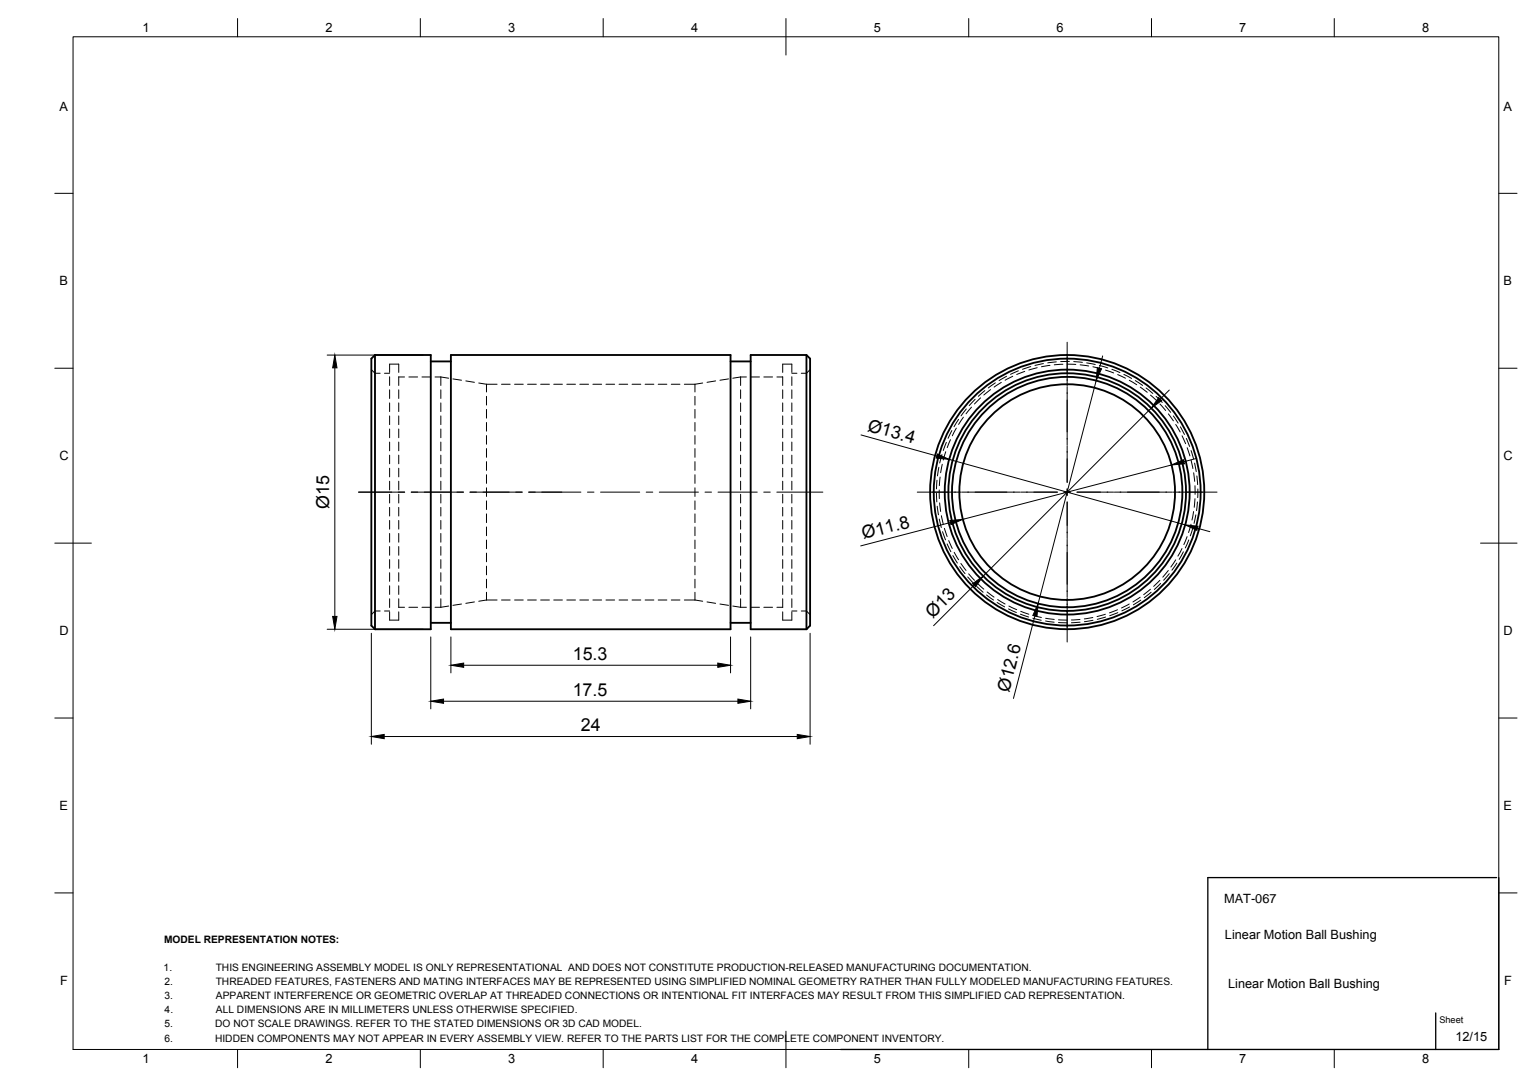
ISO-10303-21;
HEADER;
/* Generated by software containing ST-Developer
 * from STEP Tools, Inc. (www.steptools.com) 
 */

FILE_DESCRIPTION(
/* description */ ('CAx-IF Rec.Pracs.---Representation and Presentation of Product Manufa
cturing Information (PMI)---4.0---2014-10-13'),
/* implementation_level */ '2;1');

FILE_NAME(
/* name */ 'Linear Motion Ball Bushing.step',
/* time_stamp */ '2026-10-24T16:02:03-07:00',
/* author */ (''),
/* organization */ (''),
/* preprocessor_version */ 'ST-DEVELOPER v20.2',
/* originating_system */ 'Autodesk Translation Framework v15.17.0.0',
/* authorisation */ '');

FILE_SCHEMA (('AP242_MANAGED_MODEL_BASED_3D_ENGINEERING_MIM_LF { 1 0 10303 442 2 1 4 }'));
ENDSEC;

DATA;
#10=MECHANICAL_DESIGN_GEOMETRIC_PRESENTATION_REPRESENTATION('',(#356),#6348);
#315=CONICAL_SURFACE('',#3805,0.0066,0.785398163397459);
#316=CONICAL_SURFACE('',#3813,0.0074,0.785398163397448);
#317=CONICAL_SURFACE('',#3818,0.0066,0.785398163397459);
#318=CONICAL_SURFACE('',#3826,0.0074,0.785398163397448);
#319=CONICAL_SURFACE('',#3839,0.0061,0.158655262186402);
#320=CONICAL_SURFACE('',#3843,0.0061,0.158655262186402);
#334=SHAPE_REPRESENTATION_RELATIONSHIP('SRR','None',#6496,#345);
#345=ADVANCED_BREP_SHAPE_REPRESENTATION('',(#367),#6344);
#356=STYLED_ITEM('',(#6603),#367);
#367=MANIFOLD_SOLID_BREP('Body1',#3395);
#446=CYLINDRICAL_SURFACE('',#3811,0.0065);
#447=CYLINDRICAL_SURFACE('',#3816,0.0075);
#448=CYLINDRICAL_SURFACE('',#3824,0.0065);
#449=CYLINDRICAL_SURFACE('',#3829,0.0075);
#450=CYLINDRICAL_SURFACE('',#3833,0.00700000010430813);
#451=CYLINDRICAL_SURFACE('',#3837,0.0063);
#452=CYLINDRICAL_SURFACE('',#3841,0.0059);
#453=CYLINDRICAL_SURFACE('',#3845,0.0063);
#454=CYLINDRICAL_SURFACE('',#3849,0.00700000010430813);
#455=CYLINDRICAL_SURFACE('',#3854,0.00715);
#456=CYLINDRICAL_SURFACE('',#3858,0.0075);
#457=CYLINDRICAL_SURFACE('',#3862,0.00715);
#488=FACE_BOUND('',#1016,.T.);
#489=FACE_BOUND('',#1022,.T.);
#490=FACE_BOUND('',#1027,.T.);
#491=FACE_BOUND('',#1030,.T.);
#492=FACE_BOUND('',#1037,.T.);
#493=FACE_BOUND('',#1040,.T.);
#494=FACE_BOUND('',#1042,.T.);
#495=FACE_BOUND('',#1045,.T.);
#496=FACE_BOUND('',#1048,.T.);
#497=FACE_BOUND('',#1051,.T.);
#644=CIRCLE('',#3806,0.00650000000001);
#645=CIRCLE('',#3807,0.00670000000001);
#646=CIRCLE('',#3808,0.00650000000001);
#647=CIRCLE('',#3810,0.00730000000001);
#648=CIRCLE('',#3812,0.00650000000001);
#649=CIRCLE('',#3814,0.00750000000001);
#650=CIRCLE('',#3815,0.00750000000001);
#651=CIRCLE('',#3817,0.00750000000001);
#652=CIRCLE('',#3819,0.00650000000001);
#653=CIRCLE('',#3820,0.00670000000001);
#654=CIRCLE('',#3821,0.00650000000001);
#655=CIRCLE('',#3823,0.00730000000001);
#656=CIRCLE('',#3825,0.00650000000001);
#657=CIRCLE('',#3827,0.00750000000001);
#658=CIRCLE('',#3828,0.00750000000001);
#659=CIRCLE('',#3830,0.00750000000001);
#660=CIRCLE('',#3832,0.00700000010431813);
#661=CIRCLE('',#3834,0.00700000010431813);
#662=CIRCLE('',#3836,0.00630000000001);
#663=CIRCLE('',#3838,0.00630000000001);
#664=CIRCLE('',#3840,0.00590000000001);
#665=CIRCLE('',#3842,0.00590000000001);
#666=CIRCLE('',#3844,0.00630000000001);
#667=CIRCLE('',#3846,0.00630000000001);
#668=CIRCLE('',#3848,0.00700000010431813);
#669=CIRCLE('',#3850,0.00700000010431813);
#670=CIRCLE('',#3853,0.00715000000001);
#671=CIRCLE('',#3855,0.00715000000001);
#672=CIRCLE('',#3857,0.00750000000001);
#673=CIRCLE('',#3859,0.00750000000001);
#674=CIRCLE('',#3861,0.00715000000001);
#675=CIRCLE('',#3863,0.00715000000001);
#819=FACE_OUTER_BOUND('',#1014,.T.);
#820=FACE_OUTER_BOUND('',#1015,.T.);
#821=FACE_OUTER_BOUND('',#1017,.T.);
#822=FACE_OUTER_BOUND('',#1018,.T.);
#823=FACE_OUTER_BOUND('',#1019,.T.);
#824=FACE_OUTER_BOUND('',#1020,.T.);
#825=FACE_OUTER_BOUND('',#1021,.T.);
#826=FACE_OUTER_BOUND('',#1023,.T.);
#827=FACE_OUTER_BOUND('',#1024,.T.);
#828=FACE_OUTER_BOUND('',#1025,.T.);
#829=FACE_OUTER_BOUND('',#1026,.T.);
#830=FACE_OUTER_BOUND('',#1028,.T.);
#831=FACE_OUTER_BOUND('',#1029,.T.);
#832=FACE_OUTER_BOUND('',#1031,.T.);
#833=FACE_OUTER_BOUND('',#1032,.T.);
#834=FACE_OUTER_BOUND('',#1033,.T.);
#835=FACE_OUTER_BOUND('',#1034,.T.);
#836=FACE_OUTER_BOUND('',#1035,.T.);
#837=FACE_OUTER_BOUND('',#1036,.T.);
#838=FACE_OUTER_BOUND('',#1038,.T.);
#839=FACE_OUTER_BOUND('',#1039,.T.);
#840=FACE_OUTER_BOUND('',#1041,.T.);
#841=FACE_OUTER_BOUND('',#1043,.T.);
#842=FACE_OUTER_BOUND('',#1044,.T.);
#843=FACE_OUTER_BOUND('',#1046,.T.);
#844=FACE_OUTER_BOUND('',#1047,.T.);
#845=FACE_OUTER_BOUND('',#1049,.T.);
#846=FACE_OUTER_BOUND('',#1050,.T.);
#1014=EDGE_LOOP('',(#2981,#2982,#2983,#2984,#2985));
#1015=EDGE_LOOP('',(#2986));
#1016=EDGE_LOOP('',(#2987));
#1017=EDGE_LOOP('',(#2988,#2989,#2990,#2991,#2992));
#1018=EDGE_LOOP('',(#2993,#2994,#2995,#2996,#2997));
#1019=EDGE_LOOP('',(#2998,#2999,#3000,#3001,#3002));
#1020=EDGE_LOOP('',(#3003,#3004,#3005,#3006,#3007));
#1021=EDGE_LOOP('',(#3008));
#1022=EDGE_LOOP('',(#3009));
#1023=EDGE_LOOP('',(#3010,#3011,#3012,#3013,#3014));
#1024=EDGE_LOOP('',(#3015,#3016,#3017,#3018,#3019));
#1025=EDGE_LOOP('',(#3020,#3021,#3022,#3023,#3024));
#1026=EDGE_LOOP('',(#3025));
#1027=EDGE_LOOP('',(#3026));
#1028=EDGE_LOOP('',(#3027,#3028,#3029,#3030));
#1029=EDGE_LOOP('',(#3031));
#1030=EDGE_LOOP('',(#3032));
#1031=EDGE_LOOP('',(#3033,#3034,#3035,#3036));
#1032=EDGE_LOOP('',(#3037,#3038,#3039,#3040));
#1033=EDGE_LOOP('',(#3041,#3042,#3043,#3044));
#1034=EDGE_LOOP('',(#3045,#3046,#3047,#3048));
#1035=EDGE_LOOP('',(#3049,#3050,#3051,#3052));
#1036=EDGE_LOOP('',(#3053));
#1037=EDGE_LOOP('',(#3054));
#1038=EDGE_LOOP('',(#3055,#3056,#3057,#3058));
#1039=EDGE_LOOP('',(#3059));
#1040=EDGE_LOOP('',(#3060));
#1041=EDGE_LOOP('',(#3061));
#1042=EDGE_LOOP('',(#3062));
#1043=EDGE_LOOP('',(#3063,#3064,#3065,#3066));
#1044=EDGE_LOOP('',(#3067));
#1045=EDGE_LOOP('',(#3068));
#1046=EDGE_LOOP('',(#3069,#3070,#3071,#3072));
#1047=EDGE_LOOP('',(#3073));
#1048=EDGE_LOOP('',(#3074));
#1049=EDGE_LOOP('',(#3075,#3076,#3077,#3078));
#1050=EDGE_LOOP('',(#3079));
#1051=EDGE_LOOP('',(#3080));
#1283=LINE('',#6051,#1516);
#1284=LINE('',#6059,#1517);
#1285=LINE('',#6065,#1518);
#1286=LINE('',#6070,#1519);
#1287=LINE('',#6076,#1520);
#1288=LINE('',#6085,#1521);
#1289=LINE('',#6090,#1522);
#1290=LINE('',#6094,#1523);
#1291=LINE('',#6102,#1524);
#1292=LINE('',#6109,#1525);
#1293=LINE('',#6113,#1526);
#1294=LINE('',#6117,#1527);
#1295=LINE('',#6120,#1528);
#1296=LINE('',#6125,#1529);
#1297=LINE('',#6132,#1530);
#1298=LINE('',#6140,#1531);
#1299=LINE('',#6147,#1532);
#1300=LINE('',#6154,#1533);
#1516=VECTOR('',#4757,0.0066);
#1517=VECTOR('',#4768,0.0065);
#1518=VECTOR('',#4775,0.0074);
#1519=VECTOR('',#4782,0.0075);
#1520=VECTOR('',#4787,0.0066);
#1521=VECTOR('',#4800,0.0065);
#1522=VECTOR('',#4805,0.0074);
#1523=VECTOR('',#4810,0.0075);
#1524=VECTOR('',#4821,0.00700000010430813);
#1525=VECTOR('',#4830,0.0063);
#1526=VECTOR('',#4835,0.0061);
#1527=VECTOR('',#4840,0.0059);
#1528=VECTOR('',#4843,0.0061);
#1529=VECTOR('',#4850,0.0063);
#1530=VECTOR('',#4859,0.00700000010430813);
#1531=VECTOR('',#4870,0.00715);
#1532=VECTOR('',#4879,0.0075);
#1533=VECTOR('',#4888,0.00715);
#1782=VERTEX_POINT('',#6047);
#1783=VERTEX_POINT('',#6048);
#1784=VERTEX_POINT('',#6050);
#1785=VERTEX_POINT('',#6055);
#1786=VERTEX_POINT('',#6058);
#1787=VERTEX_POINT('',#6062);
#1788=VERTEX_POINT('',#6063);
#1789=VERTEX_POINT('',#6068);
#1790=VERTEX_POINT('',#6072);
#1791=VERTEX_POINT('',#6073);
#1792=VERTEX_POINT('',#6075);
#1793=VERTEX_POINT('',#6080);
#1794=VERTEX_POINT('',#6083);
#1795=VERTEX_POINT('',#6087);
#1796=VERTEX_POINT('',#6088);
#1797=VERTEX_POINT('',#6093);
#1798=VERTEX_POINT('',#6097);
#1799=VERTEX_POINT('',#6100);
#1800=VERTEX_POINT('',#6104);
#1801=VERTEX_POINT('',#6107);
#1802=VERTEX_POINT('',#6111);
#1803=VERTEX_POINT('',#6115);
#1804=VERTEX_POINT('',#6119);
#1805=VERTEX_POINT('',#6123);
#1806=VERTEX_POINT('',#6127);
#1807=VERTEX_POINT('',#6130);
#1808=VERTEX_POINT('',#6135);
#1809=VERTEX_POINT('',#6138);
#1810=VERTEX_POINT('',#6142);
#1811=VERTEX_POINT('',#6145);
#1812=VERTEX_POINT('',#6149);
#1813=VERTEX_POINT('',#6152);
#2189=EDGE_CURVE('',#1782,#1783,#644,.T.);
#2190=EDGE_CURVE('',#1783,#1784,#1283,.T.);
#2191=EDGE_CURVE('',#1784,#1784,#645,.T.);
#2192=EDGE_CURVE('',#1783,#1782,#646,.T.);
#2193=EDGE_CURVE('',#1785,#1785,#647,.T.);
#2194=EDGE_CURVE('',#1782,#1786,#1284,.T.);
#2195=EDGE_CURVE('',#1786,#1786,#648,.T.);
#2196=EDGE_CURVE('',#1787,#1788,#649,.T.);
#2197=EDGE_CURVE('',#1788,#1785,#1285,.T.);
#2198=EDGE_CURVE('',#1788,#1787,#650,.T.);
#2199=EDGE_CURVE('',#1789,#1789,#651,.T.);
#2200=EDGE_CURVE('',#1789,#1787,#1286,.T.);
#2201=EDGE_CURVE('',#1790,#1791,#652,.T.);
#2202=EDGE_CURVE('',#1791,#1792,#1287,.T.);
#2203=EDGE_CURVE('',#1792,#1792,#653,.T.);
#2204=EDGE_CURVE('',#1791,#1790,#654,.T.);
#2205=EDGE_CURVE('',#1793,#1793,#655,.T.);
#2206=EDGE_CURVE('',#1794,#1794,#656,.T.);
#2207=EDGE_CURVE('',#1794,#1790,#1288,.T.);
#2208=EDGE_CURVE('',#1795,#1796,#657,.T.);
#2209=EDGE_CURVE('',#1796,#1793,#1289,.T.);
#2210=EDGE_CURVE('',#1796,#1795,#658,.T.);
#2211=EDGE_CURVE('',#1795,#1797,#1290,.T.);
#2212=EDGE_CURVE('',#1797,#1797,#659,.T.);
#2213=EDGE_CURVE('',#1798,#1798,#660,.T.);
#2214=EDGE_CURVE('',#1799,#1799,#661,.T.);
#2215=EDGE_CURVE('',#1799,#1798,#1291,.T.);
#2216=EDGE_CURVE('',#1800,#1800,#662,.T.);
#2217=EDGE_CURVE('',#1801,#1801,#663,.T.);
#2218=EDGE_CURVE('',#1801,#1800,#1292,.T.);
#2219=EDGE_CURVE('',#1802,#1802,#664,.T.);
#2220=EDGE_CURVE('',#1802,#1801,#1293,.T.);
#2221=EDGE_CURVE('',#1803,#1803,#665,.T.);
#2222=EDGE_CURVE('',#1803,#1802,#1294,.T.);
#2223=EDGE_CURVE('',#1803,#1804,#1295,.T.);
#2224=EDGE_CURVE('',#1804,#1804,#666,.T.);
#2225=EDGE_CURVE('',#1805,#1805,#667,.T.);
#2226=EDGE_CURVE('',#1805,#1804,#1296,.T.);
#2227=EDGE_CURVE('',#1806,#1806,#668,.T.);
#2228=EDGE_CURVE('',#1807,#1807,#669,.T.);
#2229=EDGE_CURVE('',#1807,#1806,#1297,.T.);
#2230=EDGE_CURVE('',#1808,#1808,#670,.T.);
#2231=EDGE_CURVE('',#1809,#1809,#671,.T.);
#2232=EDGE_CURVE('',#1809,#1808,#1298,.T.);
#2233=EDGE_CURVE('',#1810,#1810,#672,.T.);
#2234=EDGE_CURVE('',#1811,#1811,#673,.T.);
#2235=EDGE_CURVE('',#1811,#1810,#1299,.T.);
#2236=EDGE_CURVE('',#1812,#1812,#674,.T.);
#2237=EDGE_CURVE('',#1813,#1813,#675,.T.);
#2238=EDGE_CURVE('',#1813,#1812,#1300,.T.);
#2981=ORIENTED_EDGE('',*,*,#2189,.T.);
#2982=ORIENTED_EDGE('',*,*,#2190,.T.);
#2983=ORIENTED_EDGE('',*,*,#2191,.T.);
#2984=ORIENTED_EDGE('',*,*,#2190,.F.);
#2985=ORIENTED_EDGE('',*,*,#2192,.T.);
#2986=ORIENTED_EDGE('',*,*,#2193,.F.);
#2987=ORIENTED_EDGE('',*,*,#2191,.F.);
#2988=ORIENTED_EDGE('',*,*,#2189,.F.);
#2989=ORIENTED_EDGE('',*,*,#2194,.T.);
#2990=ORIENTED_EDGE('',*,*,#2195,.T.);
#2991=ORIENTED_EDGE('',*,*,#2194,.F.);
#2992=ORIENTED_EDGE('',*,*,#2192,.F.);
#2993=ORIENTED_EDGE('',*,*,#2196,.T.);
#2994=ORIENTED_EDGE('',*,*,#2197,.T.);
#2995=ORIENTED_EDGE('',*,*,#2193,.T.);
#2996=ORIENTED_EDGE('',*,*,#2197,.F.);
#2997=ORIENTED_EDGE('',*,*,#2198,.T.);
#2998=ORIENTED_EDGE('',*,*,#2199,.F.);
#2999=ORIENTED_EDGE('',*,*,#2200,.T.);
#3000=ORIENTED_EDGE('',*,*,#2198,.F.);
#3001=ORIENTED_EDGE('',*,*,#2196,.F.);
#3002=ORIENTED_EDGE('',*,*,#2200,.F.);
#3003=ORIENTED_EDGE('',*,*,#2201,.T.);
#3004=ORIENTED_EDGE('',*,*,#2202,.T.);
#3005=ORIENTED_EDGE('',*,*,#2203,.T.);
#3006=ORIENTED_EDGE('',*,*,#2202,.F.);
#3007=ORIENTED_EDGE('',*,*,#2204,.T.);
#3008=ORIENTED_EDGE('',*,*,#2205,.F.);
#3009=ORIENTED_EDGE('',*,*,#2203,.F.);
#3010=ORIENTED_EDGE('',*,*,#2206,.F.);
#3011=ORIENTED_EDGE('',*,*,#2207,.T.);
#3012=ORIENTED_EDGE('',*,*,#2204,.F.);
#3013=ORIENTED_EDGE('',*,*,#2201,.F.);
#3014=ORIENTED_EDGE('',*,*,#2207,.F.);
#3015=ORIENTED_EDGE('',*,*,#2208,.T.);
#3016=ORIENTED_EDGE('',*,*,#2209,.T.);
#3017=ORIENTED_EDGE('',*,*,#2205,.T.);
#3018=ORIENTED_EDGE('',*,*,#2209,.F.);
#3019=ORIENTED_EDGE('',*,*,#2210,.T.);
#3020=ORIENTED_EDGE('',*,*,#2208,.F.);
#3021=ORIENTED_EDGE('',*,*,#2211,.T.);
#3022=ORIENTED_EDGE('',*,*,#2212,.T.);
#3023=ORIENTED_EDGE('',*,*,#2211,.F.);
#3024=ORIENTED_EDGE('',*,*,#2210,.F.);
#3025=ORIENTED_EDGE('',*,*,#2213,.F.);
#3026=ORIENTED_EDGE('',*,*,#2206,.T.);
#3027=ORIENTED_EDGE('',*,*,#2214,.F.);
#3028=ORIENTED_EDGE('',*,*,#2215,.T.);
#3029=ORIENTED_EDGE('',*,*,#2213,.T.);
#3030=ORIENTED_EDGE('',*,*,#2215,.F.);
#3031=ORIENTED_EDGE('',*,*,#2214,.T.);
#3032=ORIENTED_EDGE('',*,*,#2216,.F.);
#3033=ORIENTED_EDGE('',*,*,#2217,.F.);
#3034=ORIENTED_EDGE('',*,*,#2218,.T.);
#3035=ORIENTED_EDGE('',*,*,#2216,.T.);
#3036=ORIENTED_EDGE('',*,*,#2218,.F.);
#3037=ORIENTED_EDGE('',*,*,#2219,.F.);
#3038=ORIENTED_EDGE('',*,*,#2220,.T.);
#3039=ORIENTED_EDGE('',*,*,#2217,.T.);
#3040=ORIENTED_EDGE('',*,*,#2220,.F.);
#3041=ORIENTED_EDGE('',*,*,#2221,.F.);
#3042=ORIENTED_EDGE('',*,*,#2222,.T.);
#3043=ORIENTED_EDGE('',*,*,#2219,.T.);
#3044=ORIENTED_EDGE('',*,*,#2222,.F.);
#3045=ORIENTED_EDGE('',*,*,#2221,.T.);
#3046=ORIENTED_EDGE('',*,*,#2223,.T.);
#3047=ORIENTED_EDGE('',*,*,#2224,.F.);
#3048=ORIENTED_EDGE('',*,*,#2223,.F.);
#3049=ORIENTED_EDGE('',*,*,#2225,.F.);
#3050=ORIENTED_EDGE('',*,*,#2226,.T.);
#3051=ORIENTED_EDGE('',*,*,#2224,.T.);
#3052=ORIENTED_EDGE('',*,*,#2226,.F.);
#3053=ORIENTED_EDGE('',*,*,#2227,.F.);
#3054=ORIENTED_EDGE('',*,*,#2225,.T.);
#3055=ORIENTED_EDGE('',*,*,#2228,.F.);
#3056=ORIENTED_EDGE('',*,*,#2229,.T.);
#3057=ORIENTED_EDGE('',*,*,#2227,.T.);
#3058=ORIENTED_EDGE('',*,*,#2229,.F.);
#3059=ORIENTED_EDGE('',*,*,#2228,.T.);
#3060=ORIENTED_EDGE('',*,*,#2195,.F.);
#3061=ORIENTED_EDGE('',*,*,#2199,.T.);
#3062=ORIENTED_EDGE('',*,*,#2230,.F.);
#3063=ORIENTED_EDGE('',*,*,#2231,.F.);
#3064=ORIENTED_EDGE('',*,*,#2232,.T.);
#3065=ORIENTED_EDGE('',*,*,#2230,.T.);
#3066=ORIENTED_EDGE('',*,*,#2232,.F.);
#3067=ORIENTED_EDGE('',*,*,#2233,.F.);
#3068=ORIENTED_EDGE('',*,*,#2231,.T.);
#3069=ORIENTED_EDGE('',*,*,#2234,.F.);
#3070=ORIENTED_EDGE('',*,*,#2235,.T.);
#3071=ORIENTED_EDGE('',*,*,#2233,.T.);
#3072=ORIENTED_EDGE('',*,*,#2235,.F.);
#3073=ORIENTED_EDGE('',*,*,#2234,.T.);
#3074=ORIENTED_EDGE('',*,*,#2236,.F.);
#3075=ORIENTED_EDGE('',*,*,#2237,.F.);
#3076=ORIENTED_EDGE('',*,*,#2238,.T.);
#3077=ORIENTED_EDGE('',*,*,#2236,.T.);
#3078=ORIENTED_EDGE('',*,*,#2238,.F.);
#3079=ORIENTED_EDGE('',*,*,#2212,.F.);
#3080=ORIENTED_EDGE('',*,*,#2237,.T.);
#3199=PLANE('',#3809);
#3200=PLANE('',#3822);
#3201=PLANE('',#3831);
#3202=PLANE('',#3835);
#3203=PLANE('',#3847);
#3204=PLANE('',#3851);
#3205=PLANE('',#3852);
#3206=PLANE('',#3856);
#3207=PLANE('',#3860);
#3208=PLANE('',#3864);
#3342=ADVANCED_FACE('',(#819),#315,.F.);
#3343=ADVANCED_FACE('',(#820,#488),#3199,.T.);
#3344=ADVANCED_FACE('',(#821),#446,.F.);
#3345=ADVANCED_FACE('',(#822),#316,.T.);
#3346=ADVANCED_FACE('',(#823),#447,.T.);
#3347=ADVANCED_FACE('',(#824),#317,.F.);
#3348=ADVANCED_FACE('',(#825,#489),#3200,.T.);
#3349=ADVANCED_FACE('',(#826),#448,.F.);
#3350=ADVANCED_FACE('',(#827),#318,.T.);
#3351=ADVANCED_FACE('',(#828),#449,.T.);
#3352=ADVANCED_FACE('',(#829,#490),#3201,.T.);
#3353=ADVANCED_FACE('',(#830),#450,.F.);
#3354=ADVANCED_FACE('',(#831,#491),#3202,.T.);
#3355=ADVANCED_FACE('',(#832),#451,.F.);
#3356=ADVANCED_FACE('',(#833),#319,.F.);
#3357=ADVANCED_FACE('',(#834),#452,.F.);
#3358=ADVANCED_FACE('',(#835),#320,.F.);
#3359=ADVANCED_FACE('',(#836),#453,.F.);
#3360=ADVANCED_FACE('',(#837,#492),#3203,.T.);
#3361=ADVANCED_FACE('',(#838),#454,.F.);
#3362=ADVANCED_FACE('',(#839,#493),#3204,.T.);
#3363=ADVANCED_FACE('',(#840,#494),#3205,.T.);
#3364=ADVANCED_FACE('',(#841),#455,.T.);
#3365=ADVANCED_FACE('',(#842,#495),#3206,.T.);
#3366=ADVANCED_FACE('',(#843),#456,.T.);
#3367=ADVANCED_FACE('',(#844,#496),#3207,.T.);
#3368=ADVANCED_FACE('',(#845),#457,.T.);
#3369=ADVANCED_FACE('',(#846,#497),#3208,.T.);
#3395=CLOSED_SHELL('',(#3342,#3343,#3344,#3345,#3346,#3347,#3348,#3349,
#3350,#3351,#3352,#3353,#3354,#3355,#3356,#3357,#3358,#3359,#3360,#3361,
#3362,#3363,#3364,#3365,#3366,#3367,#3368,#3369));
#3804=AXIS2_PLACEMENT_3D('',#6045,#4751,#4752);
#3805=AXIS2_PLACEMENT_3D('',#6046,#4753,#4754);
#3806=AXIS2_PLACEMENT_3D('',#6049,#4755,#4756);
#3807=AXIS2_PLACEMENT_3D('',#6052,#4758,#4759);
#3808=AXIS2_PLACEMENT_3D('',#6053,#4760,#4761);
#3809=AXIS2_PLACEMENT_3D('',#6054,#4762,#4763);
#3810=AXIS2_PLACEMENT_3D('',#6056,#4764,#4765);
#3811=AXIS2_PLACEMENT_3D('',#6057,#4766,#4767);
#3812=AXIS2_PLACEMENT_3D('',#6060,#4769,#4770);
#3813=AXIS2_PLACEMENT_3D('',#6061,#4771,#4772);
#3814=AXIS2_PLACEMENT_3D('',#6064,#4773,#4774);
#3815=AXIS2_PLACEMENT_3D('',#6066,#4776,#4777);
#3816=AXIS2_PLACEMENT_3D('',#6067,#4778,#4779);
#3817=AXIS2_PLACEMENT_3D('',#6069,#4780,#4781);
#3818=AXIS2_PLACEMENT_3D('',#6071,#4783,#4784);
#3819=AXIS2_PLACEMENT_3D('',#6074,#4785,#4786);
#3820=AXIS2_PLACEMENT_3D('',#6077,#4788,#4789);
#3821=AXIS2_PLACEMENT_3D('',#6078,#4790,#4791);
#3822=AXIS2_PLACEMENT_3D('',#6079,#4792,#4793);
#3823=AXIS2_PLACEMENT_3D('',#6081,#4794,#4795);
#3824=AXIS2_PLACEMENT_3D('',#6082,#4796,#4797);
#3825=AXIS2_PLACEMENT_3D('',#6084,#4798,#4799);
#3826=AXIS2_PLACEMENT_3D('',#6086,#4801,#4802);
#3827=AXIS2_PLACEMENT_3D('',#6089,#4803,#4804);
#3828=AXIS2_PLACEMENT_3D('',#6091,#4806,#4807);
#3829=AXIS2_PLACEMENT_3D('',#6092,#4808,#4809);
#3830=AXIS2_PLACEMENT_3D('',#6095,#4811,#4812);
#3831=AXIS2_PLACEMENT_3D('',#6096,#4813,#4814);
#3832=AXIS2_PLACEMENT_3D('',#6098,#4815,#4816);
#3833=AXIS2_PLACEMENT_3D('',#6099,#4817,#4818);
#3834=AXIS2_PLACEMENT_3D('',#6101,#4819,#4820);
#3835=AXIS2_PLACEMENT_3D('',#6103,#4822,#4823);
#3836=AXIS2_PLACEMENT_3D('',#6105,#4824,#4825);
#3837=AXIS2_PLACEMENT_3D('',#6106,#4826,#4827);
#3838=AXIS2_PLACEMENT_3D('',#6108,#4828,#4829);
#3839=AXIS2_PLACEMENT_3D('',#6110,#4831,#4832);
#3840=AXIS2_PLACEMENT_3D('',#6112,#4833,#4834);
#3841=AXIS2_PLACEMENT_3D('',#6114,#4836,#4837);
#3842=AXIS2_PLACEMENT_3D('',#6116,#4838,#4839);
#3843=AXIS2_PLACEMENT_3D('',#6118,#4841,#4842);
#3844=AXIS2_PLACEMENT_3D('',#6121,#4844,#4845);
#3845=AXIS2_PLACEMENT_3D('',#6122,#4846,#4847);
#3846=AXIS2_PLACEMENT_3D('',#6124,#4848,#4849);
#3847=AXIS2_PLACEMENT_3D('',#6126,#4851,#4852);
#3848=AXIS2_PLACEMENT_3D('',#6128,#4853,#4854);
#3849=AXIS2_PLACEMENT_3D('',#6129,#4855,#4856);
#3850=AXIS2_PLACEMENT_3D('',#6131,#4857,#4858);
#3851=AXIS2_PLACEMENT_3D('',#6133,#4860,#4861);
#3852=AXIS2_PLACEMENT_3D('',#6134,#4862,#4863);
#3853=AXIS2_PLACEMENT_3D('',#6136,#4864,#4865);
#3854=AXIS2_PLACEMENT_3D('',#6137,#4866,#4867);
#3855=AXIS2_PLACEMENT_3D('',#6139,#4868,#4869);
#3856=AXIS2_PLACEMENT_3D('',#6141,#4871,#4872);
#3857=AXIS2_PLACEMENT_3D('',#6143,#4873,#4874);
#3858=AXIS2_PLACEMENT_3D('',#6144,#4875,#4876);
#3859=AXIS2_PLACEMENT_3D('',#6146,#4877,#4878);
#3860=AXIS2_PLACEMENT_3D('',#6148,#4880,#4881);
#3861=AXIS2_PLACEMENT_3D('',#6150,#4882,#4883);
#3862=AXIS2_PLACEMENT_3D('',#6151,#4884,#4885);
#3863=AXIS2_PLACEMENT_3D('',#6153,#4886,#4887);
#3864=AXIS2_PLACEMENT_3D('',#6155,#4889,#4890);
#4751=DIRECTION('axis',(0.,0.,1.));
#4752=DIRECTION('refdir',(1.,0.,0.));
#4753=DIRECTION('center_axis',(0.,-1.,0.));
#4754=DIRECTION('ref_axis',(0.,0.,-1.));
#4755=DIRECTION('center_axis',(0.,1.,0.));
#4756=DIRECTION('ref_axis',(0.,0.,-1.));
#4757=DIRECTION('',(-8.65956056235503E-17,-0.70710678118654,0.707106781186555));
#4758=DIRECTION('center_axis',(0.,-1.,0.));
#4759=DIRECTION('ref_axis',(0.,0.,-1.));
#4760=DIRECTION('center_axis',(0.,1.,0.));
#4761=DIRECTION('ref_axis',(0.,0.,-1.));
#4762=DIRECTION('center_axis',(0.,-1.,0.));
#4763=DIRECTION('ref_axis',(0.,0.,-1.));
#4764=DIRECTION('center_axis',(0.,1.,0.));
#4765=DIRECTION('ref_axis',(0.,0.,-1.));
#4766=DIRECTION('center_axis',(0.,1.,0.));
#4767=DIRECTION('ref_axis',(0.,0.,1.));
#4768=DIRECTION('',(0.,1.,0.));
#4769=DIRECTION('center_axis',(0.,1.,0.));
#4770=DIRECTION('ref_axis',(1.,0.,0.));
#4771=DIRECTION('center_axis',(0.,1.,0.));
#4772=DIRECTION('ref_axis',(0.,0.,-1.));
#4773=DIRECTION('center_axis',(0.,-1.,0.));
#4774=DIRECTION('ref_axis',(0.,0.,-1.));
#4775=DIRECTION('',(-8.65956056235493E-17,-0.707106781186548,-0.707106781186547));
#4776=DIRECTION('center_axis',(0.,-1.,0.));
#4777=DIRECTION('ref_axis',(0.,0.,-1.));
#4778=DIRECTION('center_axis',(0.,1.,0.));
#4779=DIRECTION('ref_axis',(0.,0.,1.));
#4780=DIRECTION('center_axis',(0.,1.,0.));
#4781=DIRECTION('ref_axis',(1.,0.,0.));
#4782=DIRECTION('',(0.,-1.,0.));
#4783=DIRECTION('center_axis',(0.,1.,0.));
#4784=DIRECTION('ref_axis',(0.,0.,-1.));
#4785=DIRECTION('center_axis',(0.,-1.,0.));
#4786=DIRECTION('ref_axis',(0.,0.,-1.));
#4787=DIRECTION('',(8.65956056235503E-17,0.70710678118654,0.707106781186555));
#4788=DIRECTION('center_axis',(0.,1.,0.));
#4789=DIRECTION('ref_axis',(0.,0.,-1.));
#4790=DIRECTION('center_axis',(0.,-1.,0.));
#4791=DIRECTION('ref_axis',(0.,0.,-1.));
#4792=DIRECTION('center_axis',(0.,1.,0.));
#4793=DIRECTION('ref_axis',(1.,0.,0.));
#4794=DIRECTION('center_axis',(0.,-1.,0.));
#4795=DIRECTION('ref_axis',(0.,0.,-1.));
#4796=DIRECTION('center_axis',(0.,1.,0.));
#4797=DIRECTION('ref_axis',(0.,0.,1.));
#4798=DIRECTION('center_axis',(0.,1.,0.));
#4799=DIRECTION('ref_axis',(1.,0.,0.));
#4800=DIRECTION('',(0.,1.,0.));
#4801=DIRECTION('center_axis',(0.,-1.,0.));
#4802=DIRECTION('ref_axis',(0.,0.,-1.));
#4803=DIRECTION('center_axis',(0.,1.,0.));
#4804=DIRECTION('ref_axis',(0.,0.,-1.));
#4805=DIRECTION('',(8.65956056235493E-17,0.707106781186548,-0.707106781186547));
#4806=DIRECTION('center_axis',(0.,1.,0.));
#4807=DIRECTION('ref_axis',(0.,0.,-1.));
#4808=DIRECTION('center_axis',(0.,1.,0.));
#4809=DIRECTION('ref_axis',(0.,0.,1.));
#4810=DIRECTION('',(0.,-1.,0.));
#4811=DIRECTION('center_axis',(0.,1.,0.));
#4812=DIRECTION('ref_axis',(1.,0.,0.));
#4813=DIRECTION('center_axis',(0.,-1.,0.));
#4814=DIRECTION('ref_axis',(0.,0.,-1.));
#4815=DIRECTION('center_axis',(0.,1.,0.));
#4816=DIRECTION('ref_axis',(1.,0.,0.));
#4817=DIRECTION('center_axis',(0.,1.,0.));
#4818=DIRECTION('ref_axis',(0.,0.,1.));
#4819=DIRECTION('center_axis',(0.,1.,0.));
#4820=DIRECTION('ref_axis',(1.,0.,0.));
#4821=DIRECTION('',(0.,1.,0.));
#4822=DIRECTION('center_axis',(0.,1.,0.));
#4823=DIRECTION('ref_axis',(1.,0.,0.));
#4824=DIRECTION('center_axis',(0.,1.,0.));
#4825=DIRECTION('ref_axis',(1.,0.,0.));
#4826=DIRECTION('center_axis',(0.,1.,0.));
#4827=DIRECTION('ref_axis',(0.,0.,1.));
#4828=DIRECTION('center_axis',(0.,1.,0.));
#4829=DIRECTION('ref_axis',(1.,0.,0.));
#4830=DIRECTION('',(0.,1.,0.));
#4831=DIRECTION('center_axis',(0.,1.,0.));
#4832=DIRECTION('ref_axis',(0.,0.,1.));
#4833=DIRECTION('center_axis',(0.,1.,0.));
#4834=DIRECTION('ref_axis',(1.,0.,0.));
#4835=DIRECTION('',(-1.93482561475974E-17,0.987440631916705,-0.157990501106673));
#4836=DIRECTION('center_axis',(0.,1.,0.));
#4837=DIRECTION('ref_axis',(0.,0.,1.));
#4838=DIRECTION('center_axis',(0.,1.,0.));
#4839=DIRECTION('ref_axis',(1.,0.,0.));
#4840=DIRECTION('',(0.,1.,0.));
#4841=DIRECTION('center_axis',(0.,-1.,0.));
#4842=DIRECTION('ref_axis',(0.,0.,1.));
#4843=DIRECTION('',(1.93482561475974E-17,-0.987440631916705,-0.157990501106673));
#4844=DIRECTION('center_axis',(0.,1.,0.));
#4845=DIRECTION('ref_axis',(1.,0.,0.));
#4846=DIRECTION('center_axis',(0.,1.,0.));
#4847=DIRECTION('ref_axis',(0.,0.,1.));
#4848=DIRECTION('center_axis',(0.,1.,0.));
#4849=DIRECTION('ref_axis',(1.,0.,0.));
#4850=DIRECTION('',(0.,1.,0.));
#4851=DIRECTION('center_axis',(0.,-1.,0.));
#4852=DIRECTION('ref_axis',(0.,0.,-1.));
#4853=DIRECTION('center_axis',(0.,1.,0.));
#4854=DIRECTION('ref_axis',(1.,0.,0.));
#4855=DIRECTION('center_axis',(0.,1.,0.));
#4856=DIRECTION('ref_axis',(0.,0.,1.));
#4857=DIRECTION('center_axis',(0.,1.,0.));
#4858=DIRECTION('ref_axis',(1.,0.,0.));
#4859=DIRECTION('',(0.,1.,0.));
#4860=DIRECTION('center_axis',(0.,1.,0.));
#4861=DIRECTION('ref_axis',(1.,0.,0.));
#4862=DIRECTION('center_axis',(0.,1.,0.));
#4863=DIRECTION('ref_axis',(1.,0.,0.));
#4864=DIRECTION('center_axis',(0.,1.,0.));
#4865=DIRECTION('ref_axis',(1.,0.,0.));
#4866=DIRECTION('center_axis',(0.,1.,0.));
#4867=DIRECTION('ref_axis',(0.,0.,1.));
#4868=DIRECTION('center_axis',(0.,1.,0.));
#4869=DIRECTION('ref_axis',(1.,0.,0.));
#4870=DIRECTION('',(0.,-1.,0.));
#4871=DIRECTION('center_axis',(0.,-1.,0.));
#4872=DIRECTION('ref_axis',(0.,0.,-1.));
#4873=DIRECTION('center_axis',(0.,1.,0.));
#4874=DIRECTION('ref_axis',(1.,0.,0.));
#4875=DIRECTION('center_axis',(0.,1.,0.));
#4876=DIRECTION('ref_axis',(0.,0.,1.));
#4877=DIRECTION('center_axis',(0.,1.,0.));
#4878=DIRECTION('ref_axis',(1.,0.,0.));
#4879=DIRECTION('',(0.,-1.,0.));
#4880=DIRECTION('center_axis',(0.,1.,0.));
#4881=DIRECTION('ref_axis',(1.,0.,0.));
#4882=DIRECTION('center_axis',(0.,1.,0.));
#4883=DIRECTION('ref_axis',(1.,0.,0.));
#4884=DIRECTION('center_axis',(0.,1.,0.));
#4885=DIRECTION('ref_axis',(0.,0.,1.));
#4886=DIRECTION('center_axis',(0.,1.,0.));
#4887=DIRECTION('ref_axis',(1.,0.,0.));
#4888=DIRECTION('',(0.,-1.,0.));
#4889=DIRECTION('center_axis',(0.,-1.,0.));
#4890=DIRECTION('ref_axis',(0.,0.,-1.));
#6045=CARTESIAN_POINT('',(0.,0.,0.));
#6046=CARTESIAN_POINT('Origin',(0.,-0.0119,0.));
#6047=CARTESIAN_POINT('',(0.,-0.01180000000001,-0.00650000000001));
#6048=CARTESIAN_POINT('',(-7.96020419447004E-19,-0.01180000000001,0.00650000000001));
#6049=CARTESIAN_POINT('Origin',(0.,-0.01180000000001,0.));
#6050=CARTESIAN_POINT('',(-8.20513355429951E-19,-0.01200000000001,0.00670000000001));
#6051=CARTESIAN_POINT('',(-8.08266887437253E-19,-0.0119,0.0066));
#6052=CARTESIAN_POINT('Origin',(0.,-0.01200000000001,0.));
#6053=CARTESIAN_POINT('Origin',(0.,-0.01180000000001,0.));
#6054=CARTESIAN_POINT('Origin',(0.,-0.012,0.0075));
#6055=CARTESIAN_POINT('',(8.93992163377568E-19,-0.012,0.0073));
#6056=CARTESIAN_POINT('Origin',(0.,-0.01200000000001,0.));
#6057=CARTESIAN_POINT('Origin',(0.,-0.0115000000819564,0.));
#6058=CARTESIAN_POINT('',(-7.9602041944578E-19,-0.0110000001639228,-0.0065));
#6059=CARTESIAN_POINT('',(-7.9602041944578E-19,-0.0115000000819564,-0.0065));
#6060=CARTESIAN_POINT('Origin',(0.,-0.0110000001639228,0.));
#6061=CARTESIAN_POINT('Origin',(0.,-0.0119,0.));
#6062=CARTESIAN_POINT('',(0.,-0.01180000000001,-0.00750000000001));
#6063=CARTESIAN_POINT('',(9.18485099360515E-19,-0.0118,0.0075));
#6064=CARTESIAN_POINT('Origin',(0.,-0.01180000000001,0.));
#6065=CARTESIAN_POINT('',(9.06238631369041E-19,-0.0119,0.0074));
#6066=CARTESIAN_POINT('Origin',(0.,-0.01180000000001,0.));
#6067=CARTESIAN_POINT('Origin',(0.,-0.010375,0.));
#6068=CARTESIAN_POINT('',(-9.18485099360515E-19,-0.00875000000001,-0.0075));
#6069=CARTESIAN_POINT('Origin',(0.,-0.00875000000001,0.));
#6070=CARTESIAN_POINT('',(-9.18485099360515E-19,-0.010375,-0.0075));
#6071=CARTESIAN_POINT('Origin',(0.,0.0119,0.));
#6072=CARTESIAN_POINT('',(0.,0.01180000000001,-0.00650000000001));
#6073=CARTESIAN_POINT('',(7.96020419447004E-19,0.01180000000001,0.00650000000001));
#6074=CARTESIAN_POINT('Origin',(0.,0.01180000000001,0.));
#6075=CARTESIAN_POINT('',(8.20513355429951E-19,0.01200000000001,0.00670000000001));
#6076=CARTESIAN_POINT('',(8.08266887437253E-19,0.0119,0.0066));
#6077=CARTESIAN_POINT('Origin',(0.,0.01200000000001,0.));
#6078=CARTESIAN_POINT('Origin',(0.,0.01180000000001,0.));
#6079=CARTESIAN_POINT('Origin',(0.,0.012,0.0065));
#6080=CARTESIAN_POINT('',(-8.93992163377568E-19,0.012,0.0073));
#6081=CARTESIAN_POINT('Origin',(0.,0.01200000000001,0.));
#6082=CARTESIAN_POINT('Origin',(0.,0.0115000000819564,0.));
#6083=CARTESIAN_POINT('',(-7.9602041944578E-19,0.0110000001639228,-0.0065));
#6084=CARTESIAN_POINT('Origin',(0.,0.0110000001639228,0.));
#6085=CARTESIAN_POINT('',(-7.9602041944578E-19,0.0115000000819564,-0.0065));
#6086=CARTESIAN_POINT('Origin',(0.,0.0119,0.));
#6087=CARTESIAN_POINT('',(0.,0.01180000000001,-0.00750000000001));
#6088=CARTESIAN_POINT('',(-9.18485099360515E-19,0.0118,0.0075));
#6089=CARTESIAN_POINT('Origin',(0.,0.01180000000001,0.));
#6090=CARTESIAN_POINT('',(-9.06238631369041E-19,0.0119,0.0074));
#6091=CARTESIAN_POINT('Origin',(0.,0.01180000000001,0.));
#6092=CARTESIAN_POINT('Origin',(0.,0.010375,0.));
#6093=CARTESIAN_POINT('',(-9.18485099360515E-19,0.00875000000001,-0.0075));
#6094=CARTESIAN_POINT('',(-9.18485099360515E-19,0.010375,-0.0075));
#6095=CARTESIAN_POINT('Origin',(0.,0.00875000000001,0.));
#6096=CARTESIAN_POINT('Origin',(0.,0.0110000001639128,0.00700000010430813));
#6097=CARTESIAN_POINT('',(-8.57252772177209E-19,0.0110000001639228,-0.00700000010430813));
#6098=CARTESIAN_POINT('Origin',(0.,0.0110000001639228,0.));
#6099=CARTESIAN_POINT('Origin',(0.,0.0107500001601875,0.));
#6100=CARTESIAN_POINT('',(-8.57252772177209E-19,0.0105000001564722,-0.00700000010430813));
#6101=CARTESIAN_POINT('Origin',(0.,0.0105000001564722,0.));
#6102=CARTESIAN_POINT('',(-8.57252772177209E-19,0.0107500001601875,-0.00700000010430813));
#6103=CARTESIAN_POINT('Origin',(0.,0.0105000001564622,0.0063));
#6104=CARTESIAN_POINT('',(-7.71527483462833E-19,0.0105000001564722,-0.0063));
#6105=CARTESIAN_POINT('Origin',(0.,0.0105000001564722,0.));
#6106=CARTESIAN_POINT('Origin',(0.,0.0093500000782311,0.));
#6107=CARTESIAN_POINT('',(-7.71527483462833E-19,0.00820000000001,-0.0063));
#6108=CARTESIAN_POINT('Origin',(0.,0.00820000000001,0.));
#6109=CARTESIAN_POINT('',(-7.71527483462833E-19,0.0093500000782311,-0.0063));
#6110=CARTESIAN_POINT('Origin',(0.,0.00695,0.));
#6111=CARTESIAN_POINT('',(-7.2254161149716E-19,0.00570000000001131,-0.00590000000000181));
#6112=CARTESIAN_POINT('Origin',(0.,0.00570000000001,0.));
#6113=CARTESIAN_POINT('',(-7.47034547479885E-19,0.00695,-0.0061));
#6114=CARTESIAN_POINT('Origin',(0.,0.,0.));
#6115=CARTESIAN_POINT('',(-7.22541611496938E-19,-0.00570000000001,-0.0059));
#6116=CARTESIAN_POINT('Origin',(0.,-0.00570000000001,0.));
#6117=CARTESIAN_POINT('',(-7.22541611496938E-19,0.,-0.0059));
#6118=CARTESIAN_POINT('Origin',(0.,-0.00695,0.));
#6119=CARTESIAN_POINT('',(7.71527483463054E-19,-0.00820000000001131,-0.00630000000000181));
#6120=CARTESIAN_POINT('',(7.47034547479885E-19,-0.00695,-0.0061));
#6121=CARTESIAN_POINT('Origin',(0.,-0.00820000000001,0.));
#6122=CARTESIAN_POINT('Origin',(0.,-0.0093500000782311,0.));
#6123=CARTESIAN_POINT('',(-7.71527483462833E-19,-0.0105000001564722,-0.0063));
#6124=CARTESIAN_POINT('Origin',(0.,-0.0105000001564722,0.));
#6125=CARTESIAN_POINT('',(-7.71527483462833E-19,-0.0093500000782311,-0.0063));
#6126=CARTESIAN_POINT('Origin',(0.,-0.0105000001564622,0.00700000010430813));
#6127=CARTESIAN_POINT('',(-8.57252772177209E-19,-0.0105000001564722,-0.00700000010430813));
#6128=CARTESIAN_POINT('Origin',(0.,-0.0105000001564722,0.));
#6129=CARTESIAN_POINT('Origin',(0.,-0.0107500001601875,0.));
#6130=CARTESIAN_POINT('',(-8.57252772177209E-19,-0.0110000001639228,-0.00700000010430813));
#6131=CARTESIAN_POINT('Origin',(0.,-0.0110000001639228,0.));
#6132=CARTESIAN_POINT('',(-8.57252772177209E-19,-0.0107500001601875,-0.00700000010430813));
#6133=CARTESIAN_POINT('Origin',(0.,-0.0110000001639128,0.0065));
#6134=CARTESIAN_POINT('Origin',(0.,-0.00875,0.00715));
#6135=CARTESIAN_POINT('',(-8.75622461390357E-19,-0.00875000000001,-0.00715));
#6136=CARTESIAN_POINT('Origin',(0.,-0.00875000000001,0.));
#6137=CARTESIAN_POINT('Origin',(0.,-0.0082,0.));
#6138=CARTESIAN_POINT('',(-8.75622461390357E-19,-0.00765000000001,-0.00715));
#6139=CARTESIAN_POINT('Origin',(0.,-0.00765000000001,0.));
#6140=CARTESIAN_POINT('',(-8.75622461390357E-19,-0.0082,-0.00715));
#6141=CARTESIAN_POINT('Origin',(0.,-0.00765,0.0075));
#6142=CARTESIAN_POINT('',(-9.18485099360515E-19,-0.00765000000001,-0.0075));
#6143=CARTESIAN_POINT('Origin',(0.,-0.00765000000001,0.));
#6144=CARTESIAN_POINT('Origin',(0.,0.,0.));
#6145=CARTESIAN_POINT('',(-9.18485099360515E-19,0.00765000000001,-0.0075));
#6146=CARTESIAN_POINT('Origin',(0.,0.00765000000001,0.));
#6147=CARTESIAN_POINT('',(-9.18485099360515E-19,0.,-0.0075));
#6148=CARTESIAN_POINT('Origin',(0.,0.00765,0.00715));
#6149=CARTESIAN_POINT('',(-8.75622461390357E-19,0.00765000000001,-0.00715));
#6150=CARTESIAN_POINT('Origin',(0.,0.00765000000001,0.));
#6151=CARTESIAN_POINT('Origin',(0.,0.0082,0.));
#6152=CARTESIAN_POINT('',(-8.75622461390357E-19,0.00875000000001,-0.00715));
#6153=CARTESIAN_POINT('Origin',(0.,0.00875000000001,0.));
#6154=CARTESIAN_POINT('',(-8.75622461390357E-19,0.0082,-0.00715));
#6155=CARTESIAN_POINT('Origin',(0.,0.00875,0.0075));
#6319=UNCERTAINTY_MEASURE_WITH_UNIT(LENGTH_MEASURE(1.E-5),#6349,
'DISTANCE_ACCURACY_VALUE',
'Maximum model space distance between geometric entities at asserted c
onnectivities');
#6323=UNCERTAINTY_MEASURE_WITH_UNIT(LENGTH_MEASURE(1.E-5),#6349,
'DISTANCE_ACCURACY_VALUE',
'Maximum model space distance between geometric entities at asserted c
onnectivities');
#6344=(
GEOMETRIC_REPRESENTATION_CONTEXT(3)
GLOBAL_UNCERTAINTY_ASSIGNED_CONTEXT((#6319))
GLOBAL_UNIT_ASSIGNED_CONTEXT((#6349,#6350,#6351))
REPRESENTATION_CONTEXT('','3D')
);
#6348=(
GEOMETRIC_REPRESENTATION_CONTEXT(3)
GLOBAL_UNCERTAINTY_ASSIGNED_CONTEXT((#6323))
GLOBAL_UNIT_ASSIGNED_CONTEXT((#6349,#6350,#6351))
REPRESENTATION_CONTEXT('','3D')
);
#6349=(
LENGTH_UNIT()
NAMED_UNIT(*)
SI_UNIT($,.METRE.)
);
#6350=(
NAMED_UNIT(*)
PLANE_ANGLE_UNIT()
SI_UNIT($,.RADIAN.)
);
#6351=(
NAMED_UNIT(*)
SI_UNIT($,.STERADIAN.)
SOLID_ANGLE_UNIT()
);
#6372=SHAPE_DEFINITION_REPRESENTATION(#6396,#6496);
#6396=PRODUCT_DEFINITION_SHAPE('',$,#6521);
#6496=SHAPE_REPRESENTATION('',(#3804),#6344);
#6500=PRODUCT_DEFINITION_CONTEXT('part definition',#6574,'design');
#6521=PRODUCT_DEFINITION('Linear Motion Ball Bushing',
'Linear Motion Ball Bushing',#6545,#6500);
#6545=PRODUCT_DEFINITION_FORMATION('',$,#6596);
#6574=APPLICATION_CONTEXT('Managed model based 3d engineering');
#6575=PRODUCT_CONTEXT('part definition',#6574,'mechanical');
#6596=PRODUCT('Linear Motion Ball Bushing','Linear Motion Ball Bushing',

'LEGAL AND USAGE DISCLAIMER: this Data/Model is provided \X2\201C\X0\A
S IS\X2\201D\X0\ for informational and representational only. It is a 
geometric approximation and is NOT engineered, certified, or guarantee
d for dimensional accuracy, exact tolerances, or production-level prec
ision. Vendor disclaims all implied warranties including fitness for a
 particular purpose. DO NOT USE FOR DIRECT PHYSICAL MANUFACTURING, AUT
OMATED PRODUCTION, OR SAFETY-CRITICAL SYSTEMS without independent engi
neering verification and resolution of any design discrepancies.',(#6575));
#6603=PRESENTATION_STYLE_ASSIGNMENT((#6609));
#6609=SURFACE_STYLE_USAGE(.BOTH.,#6615);
#6615=SURFACE_SIDE_STYLE('',(#6621));
#6621=SURFACE_STYLE_FILL_AREA(#6627);
#6627=FILL_AREA_STYLE('Opaque(137,137,137)',(#6633));
#6633=FILL_AREA_STYLE_COLOUR('Opaque(137,137,137)',#6639);
#6639=COLOUR_RGB('Opaque(137,137,137)',0.537254901960784,0.537254901960784,
0.537254901960784);
ENDSEC;
END-ISO-10303-21;
